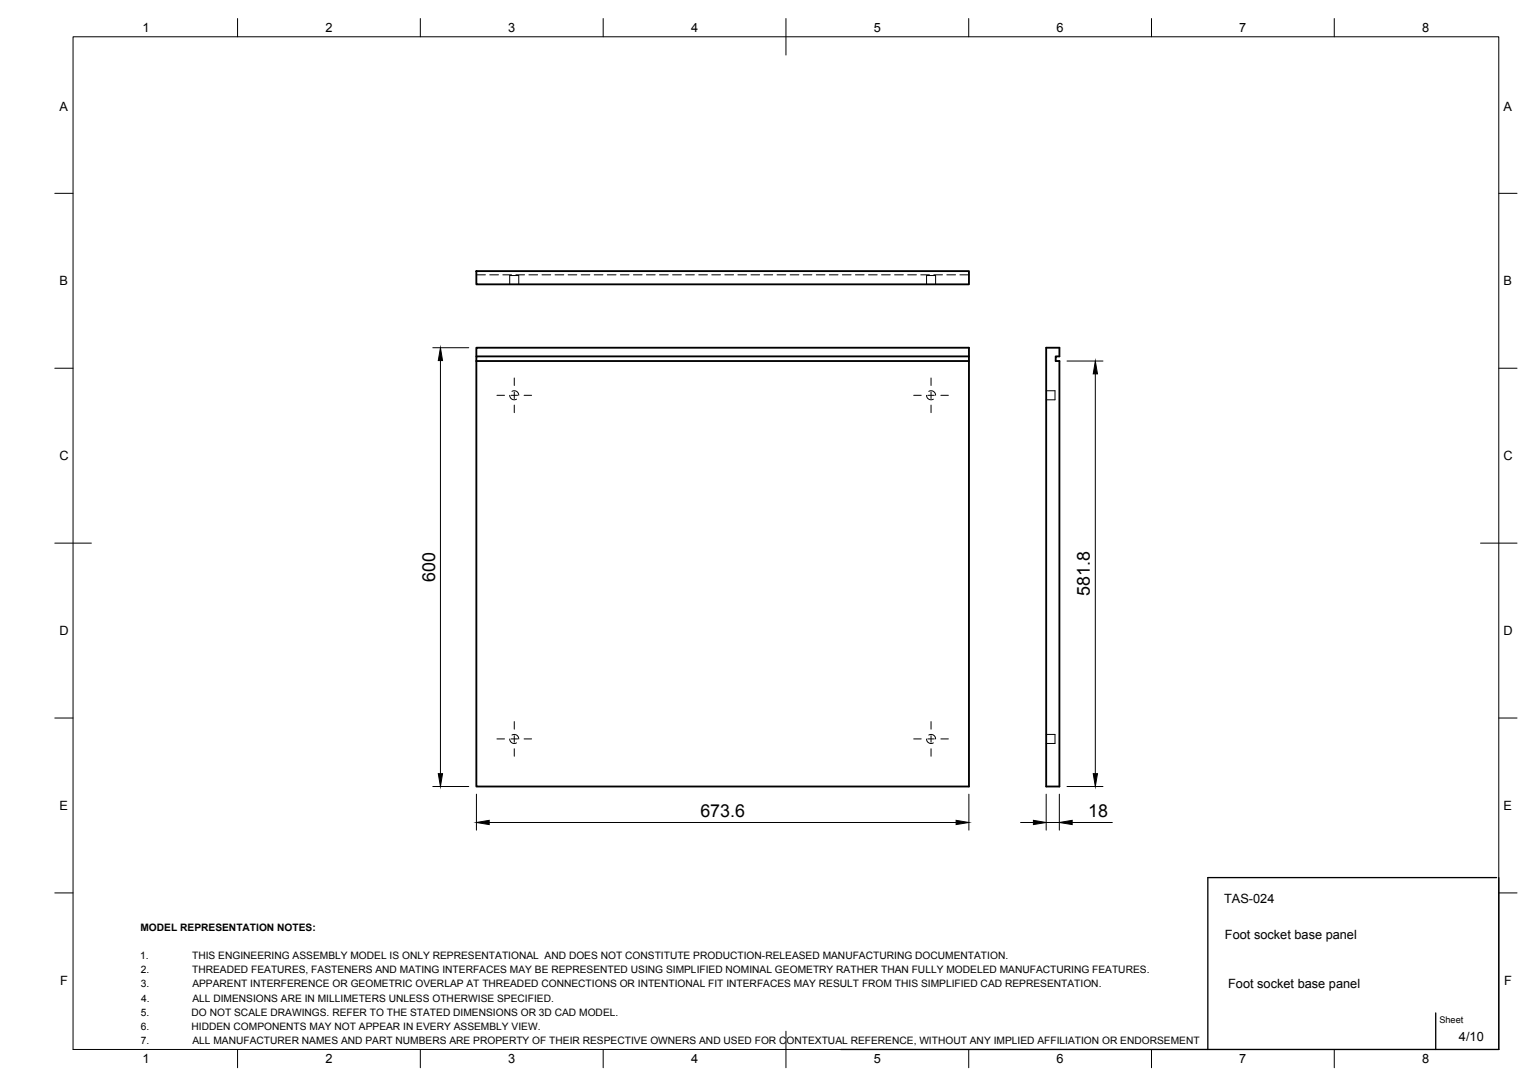
ISO-10303-21;
HEADER;
/* Generated by software containing ST-Developer
 * from STEP Tools, Inc. (www.steptools.com) 
 */

FILE_DESCRIPTION(
/* description */ (''),
/* implementation_level */ '2;1');

FILE_NAME(
/* name */ 'Foot socket base panel.step',
/* time_stamp */ '2026-11-15T17:53:25-08:00',
/* author */ (''),
/* organization */ (''),
/* preprocessor_version */ 'ST-DEVELOPER v20.2',
/* originating_system */ 'Autodesk Translation Framework v15.17.0.0',
/* authorisation */ '');

FILE_SCHEMA (('AUTOMOTIVE_DESIGN { 1 0 10303 214 3 1 1 }'));
ENDSEC;

DATA;
#10=MECHANICAL_DESIGN_GEOMETRIC_PRESENTATION_REPRESENTATION('',(#132),#2673);
#116=SHAPE_REPRESENTATION_RELATIONSHIP('SRR','None',#2724,#124);
#124=ADVANCED_BREP_SHAPE_REPRESENTATION('',(#140),#2666);
#132=STYLED_ITEM('',(#2773),#140);
#140=MANIFOLD_SOLID_BREP('Body1',#1518);
#153=FACE_BOUND('',#380,.T.);
#154=FACE_BOUND('',#381,.T.);
#155=FACE_BOUND('',#382,.T.);
#156=FACE_BOUND('',#383,.T.);
#188=PLANE('',#1666);
#189=PLANE('',#1670);
#190=PLANE('',#1674);
#191=PLANE('',#1678);
#192=PLANE('',#1679);
#193=PLANE('',#1680);
#194=PLANE('',#1681);
#195=PLANE('',#1682);
#196=PLANE('',#1683);
#197=PLANE('',#1684);
#198=PLANE('',#1685);
#199=PLANE('',#1686);
#200=PLANE('',#1687);
#201=PLANE('',#1688);
#267=FACE_OUTER_BOUND('',#362,.T.);
#268=FACE_OUTER_BOUND('',#363,.T.);
#269=FACE_OUTER_BOUND('',#364,.T.);
#270=FACE_OUTER_BOUND('',#365,.T.);
#271=FACE_OUTER_BOUND('',#366,.T.);
#272=FACE_OUTER_BOUND('',#367,.T.);
#273=FACE_OUTER_BOUND('',#368,.T.);
#274=FACE_OUTER_BOUND('',#369,.T.);
#275=FACE_OUTER_BOUND('',#370,.T.);
#276=FACE_OUTER_BOUND('',#371,.T.);
#277=FACE_OUTER_BOUND('',#372,.T.);
#278=FACE_OUTER_BOUND('',#373,.T.);
#279=FACE_OUTER_BOUND('',#374,.T.);
#280=FACE_OUTER_BOUND('',#375,.T.);
#281=FACE_OUTER_BOUND('',#376,.T.);
#282=FACE_OUTER_BOUND('',#377,.T.);
#283=FACE_OUTER_BOUND('',#378,.T.);
#284=FACE_OUTER_BOUND('',#379,.T.);
#362=EDGE_LOOP('',(#1208,#1209,#1210,#1211));
#363=EDGE_LOOP('',(#1212));
#364=EDGE_LOOP('',(#1213,#1214,#1215,#1216));
#365=EDGE_LOOP('',(#1217));
#366=EDGE_LOOP('',(#1218,#1219,#1220,#1221));
#367=EDGE_LOOP('',(#1222));
#368=EDGE_LOOP('',(#1223,#1224,#1225,#1226));
#369=EDGE_LOOP('',(#1227));
#370=EDGE_LOOP('',(#1228,#1229,#1230,#1231));
#371=EDGE_LOOP('',(#1232,#1233,#1234,#1235));
#372=EDGE_LOOP('',(#1236,#1237,#1238,#1239));
#373=EDGE_LOOP('',(#1240,#1241,#1242,#1243,#1244,#1245,#1246,#1247));
#374=EDGE_LOOP('',(#1248,#1249,#1250,#1251));
#375=EDGE_LOOP('',(#1252,#1253,#1254,#1255));
#376=EDGE_LOOP('',(#1256,#1257,#1258,#1259));
#377=EDGE_LOOP('',(#1260,#1261,#1262,#1263,#1264,#1265,#1266,#1267));
#378=EDGE_LOOP('',(#1268,#1269,#1270,#1271));
#379=EDGE_LOOP('',(#1272,#1273,#1274,#1275));
#380=EDGE_LOOP('',(#1276));
#381=EDGE_LOOP('',(#1277));
#382=EDGE_LOOP('',(#1278));
#383=EDGE_LOOP('',(#1279));
#490=LINE('',#2401,#638);
#491=LINE('',#2408,#639);
#492=LINE('',#2415,#640);
#493=LINE('',#2422,#641);
#494=LINE('',#2428,#642);
#495=LINE('',#2430,#643);
#496=LINE('',#2432,#644);
#497=LINE('',#2433,#645);
#498=LINE('',#2437,#646);
#499=LINE('',#2439,#647);
#500=LINE('',#2441,#648);
#501=LINE('',#2442,#649);
#502=LINE('',#2444,#650);
#503=LINE('',#2445,#651);
#504=LINE('',#2448,#652);
#505=LINE('',#2450,#653);
#506=LINE('',#2452,#654);
#507=LINE('',#2454,#655);
#508=LINE('',#2455,#656);
#509=LINE('',#2458,#657);
#510=LINE('',#2459,#658);
#511=LINE('',#2462,#659);
#512=LINE('',#2464,#660);
#513=LINE('',#2465,#661);
#514=LINE('',#2468,#662);
#515=LINE('',#2469,#663);
#516=LINE('',#2471,#664);
#517=LINE('',#2472,#665);
#638=VECTOR('',#1938,0.619999999999997);
#639=VECTOR('',#1947,0.62);
#640=VECTOR('',#1956,0.62);
#641=VECTOR('',#1965,0.619999999999997);
#642=VECTOR('',#1972,1.);
#643=VECTOR('',#1973,1.);
#644=VECTOR('',#1974,1.);
#645=VECTOR('',#1975,1.);
#646=VECTOR('',#1978,1.);
#647=VECTOR('',#1979,1.);
#648=VECTOR('',#1980,1.);
#649=VECTOR('',#1981,1.);
#650=VECTOR('',#1984,1.);
#651=VECTOR('',#1985,1.);
#652=VECTOR('',#1988,1.);
#653=VECTOR('',#1989,1.);
#654=VECTOR('',#1990,1.);
#655=VECTOR('',#1991,1.);
#656=VECTOR('',#1992,1.);
#657=VECTOR('',#1995,1.);
#658=VECTOR('',#1996,1.);
#659=VECTOR('',#1999,1.);
#660=VECTOR('',#2000,1.);
#661=VECTOR('',#2001,1.);
#662=VECTOR('',#2004,1.);
#663=VECTOR('',#2005,1.);
#664=VECTOR('',#2008,1.);
#665=VECTOR('',#2009,1.);
#732=CIRCLE('',#1664,0.619999999999997);
#733=CIRCLE('',#1665,0.619999999999997);
#734=CIRCLE('',#1668,0.62);
#735=CIRCLE('',#1669,0.62);
#736=CIRCLE('',#1672,0.62);
#737=CIRCLE('',#1673,0.62);
#738=CIRCLE('',#1676,0.619999999999997);
#739=CIRCLE('',#1677,0.619999999999997);
#804=VERTEX_POINT('',#2398);
#805=VERTEX_POINT('',#2400);
#806=VERTEX_POINT('',#2405);
#807=VERTEX_POINT('',#2407);
#808=VERTEX_POINT('',#2412);
#809=VERTEX_POINT('',#2414);
#810=VERTEX_POINT('',#2419);
#811=VERTEX_POINT('',#2421);
#812=VERTEX_POINT('',#2426);
#813=VERTEX_POINT('',#2427);
#814=VERTEX_POINT('',#2429);
#815=VERTEX_POINT('',#2431);
#816=VERTEX_POINT('',#2435);
#817=VERTEX_POINT('',#2436);
#818=VERTEX_POINT('',#2438);
#819=VERTEX_POINT('',#2440);
#820=VERTEX_POINT('',#2447);
#821=VERTEX_POINT('',#2449);
#822=VERTEX_POINT('',#2451);
#823=VERTEX_POINT('',#2453);
#824=VERTEX_POINT('',#2457);
#825=VERTEX_POINT('',#2461);
#826=VERTEX_POINT('',#2463);
#827=VERTEX_POINT('',#2467);
#950=EDGE_CURVE('',#804,#804,#732,.T.);
#951=EDGE_CURVE('',#804,#805,#490,.T.);
#952=EDGE_CURVE('',#805,#805,#733,.T.);
#953=EDGE_CURVE('',#806,#806,#734,.T.);
#954=EDGE_CURVE('',#806,#807,#491,.T.);
#955=EDGE_CURVE('',#807,#807,#735,.T.);
#956=EDGE_CURVE('',#808,#808,#736,.T.);
#957=EDGE_CURVE('',#808,#809,#492,.T.);
#958=EDGE_CURVE('',#809,#809,#737,.T.);
#959=EDGE_CURVE('',#810,#810,#738,.T.);
#960=EDGE_CURVE('',#810,#811,#493,.T.);
#961=EDGE_CURVE('',#811,#811,#739,.T.);
#962=EDGE_CURVE('',#812,#813,#494,.T.);
#963=EDGE_CURVE('',#814,#812,#495,.T.);
#964=EDGE_CURVE('',#815,#814,#496,.T.);
#965=EDGE_CURVE('',#813,#815,#497,.T.);
#966=EDGE_CURVE('',#816,#817,#498,.T.);
#967=EDGE_CURVE('',#818,#816,#499,.T.);
#968=EDGE_CURVE('',#819,#818,#500,.T.);
#969=EDGE_CURVE('',#817,#819,#501,.T.);
#970=EDGE_CURVE('',#815,#818,#502,.T.);
#971=EDGE_CURVE('',#819,#814,#503,.T.);
#972=EDGE_CURVE('',#820,#812,#504,.T.);
#973=EDGE_CURVE('',#821,#820,#505,.T.);
#974=EDGE_CURVE('',#821,#822,#506,.T.);
#975=EDGE_CURVE('',#822,#823,#507,.T.);
#976=EDGE_CURVE('',#817,#823,#508,.T.);
#977=EDGE_CURVE('',#813,#824,#509,.T.);
#978=EDGE_CURVE('',#824,#820,#510,.T.);
#979=EDGE_CURVE('',#822,#825,#511,.T.);
#980=EDGE_CURVE('',#825,#826,#512,.T.);
#981=EDGE_CURVE('',#823,#826,#513,.T.);
#982=EDGE_CURVE('',#827,#821,#514,.T.);
#983=EDGE_CURVE('',#827,#824,#515,.T.);
#984=EDGE_CURVE('',#826,#816,#516,.T.);
#985=EDGE_CURVE('',#825,#827,#517,.T.);
#1208=ORIENTED_EDGE('',*,*,#950,.F.);
#1209=ORIENTED_EDGE('',*,*,#951,.T.);
#1210=ORIENTED_EDGE('',*,*,#952,.T.);
#1211=ORIENTED_EDGE('',*,*,#951,.F.);
#1212=ORIENTED_EDGE('',*,*,#952,.F.);
#1213=ORIENTED_EDGE('',*,*,#953,.F.);
#1214=ORIENTED_EDGE('',*,*,#954,.T.);
#1215=ORIENTED_EDGE('',*,*,#955,.T.);
#1216=ORIENTED_EDGE('',*,*,#954,.F.);
#1217=ORIENTED_EDGE('',*,*,#955,.F.);
#1218=ORIENTED_EDGE('',*,*,#956,.F.);
#1219=ORIENTED_EDGE('',*,*,#957,.T.);
#1220=ORIENTED_EDGE('',*,*,#958,.T.);
#1221=ORIENTED_EDGE('',*,*,#957,.F.);
#1222=ORIENTED_EDGE('',*,*,#958,.F.);
#1223=ORIENTED_EDGE('',*,*,#959,.F.);
#1224=ORIENTED_EDGE('',*,*,#960,.T.);
#1225=ORIENTED_EDGE('',*,*,#961,.T.);
#1226=ORIENTED_EDGE('',*,*,#960,.F.);
#1227=ORIENTED_EDGE('',*,*,#961,.F.);
#1228=ORIENTED_EDGE('',*,*,#962,.F.);
#1229=ORIENTED_EDGE('',*,*,#963,.F.);
#1230=ORIENTED_EDGE('',*,*,#964,.F.);
#1231=ORIENTED_EDGE('',*,*,#965,.F.);
#1232=ORIENTED_EDGE('',*,*,#966,.F.);
#1233=ORIENTED_EDGE('',*,*,#967,.F.);
#1234=ORIENTED_EDGE('',*,*,#968,.F.);
#1235=ORIENTED_EDGE('',*,*,#969,.F.);
#1236=ORIENTED_EDGE('',*,*,#970,.F.);
#1237=ORIENTED_EDGE('',*,*,#964,.T.);
#1238=ORIENTED_EDGE('',*,*,#971,.F.);
#1239=ORIENTED_EDGE('',*,*,#968,.T.);
#1240=ORIENTED_EDGE('',*,*,#969,.T.);
#1241=ORIENTED_EDGE('',*,*,#971,.T.);
#1242=ORIENTED_EDGE('',*,*,#963,.T.);
#1243=ORIENTED_EDGE('',*,*,#972,.F.);
#1244=ORIENTED_EDGE('',*,*,#973,.F.);
#1245=ORIENTED_EDGE('',*,*,#974,.T.);
#1246=ORIENTED_EDGE('',*,*,#975,.T.);
#1247=ORIENTED_EDGE('',*,*,#976,.F.);
#1248=ORIENTED_EDGE('',*,*,#962,.T.);
#1249=ORIENTED_EDGE('',*,*,#977,.T.);
#1250=ORIENTED_EDGE('',*,*,#978,.T.);
#1251=ORIENTED_EDGE('',*,*,#972,.T.);
#1252=ORIENTED_EDGE('',*,*,#979,.T.);
#1253=ORIENTED_EDGE('',*,*,#980,.T.);
#1254=ORIENTED_EDGE('',*,*,#981,.F.);
#1255=ORIENTED_EDGE('',*,*,#975,.F.);
#1256=ORIENTED_EDGE('',*,*,#982,.T.);
#1257=ORIENTED_EDGE('',*,*,#973,.T.);
#1258=ORIENTED_EDGE('',*,*,#978,.F.);
#1259=ORIENTED_EDGE('',*,*,#983,.F.);
#1260=ORIENTED_EDGE('',*,*,#967,.T.);
#1261=ORIENTED_EDGE('',*,*,#984,.F.);
#1262=ORIENTED_EDGE('',*,*,#980,.F.);
#1263=ORIENTED_EDGE('',*,*,#985,.T.);
#1264=ORIENTED_EDGE('',*,*,#983,.T.);
#1265=ORIENTED_EDGE('',*,*,#977,.F.);
#1266=ORIENTED_EDGE('',*,*,#965,.T.);
#1267=ORIENTED_EDGE('',*,*,#970,.T.);
#1268=ORIENTED_EDGE('',*,*,#966,.T.);
#1269=ORIENTED_EDGE('',*,*,#976,.T.);
#1270=ORIENTED_EDGE('',*,*,#981,.T.);
#1271=ORIENTED_EDGE('',*,*,#984,.T.);
#1272=ORIENTED_EDGE('',*,*,#985,.F.);
#1273=ORIENTED_EDGE('',*,*,#979,.F.);
#1274=ORIENTED_EDGE('',*,*,#974,.F.);
#1275=ORIENTED_EDGE('',*,*,#982,.F.);
#1276=ORIENTED_EDGE('',*,*,#950,.T.);
#1277=ORIENTED_EDGE('',*,*,#953,.T.);
#1278=ORIENTED_EDGE('',*,*,#956,.T.);
#1279=ORIENTED_EDGE('',*,*,#959,.T.);
#1418=CYLINDRICAL_SURFACE('',#1663,0.619999999999997);
#1419=CYLINDRICAL_SURFACE('',#1667,0.62);
#1420=CYLINDRICAL_SURFACE('',#1671,0.62);
#1421=CYLINDRICAL_SURFACE('',#1675,0.619999999999997);
#1462=ADVANCED_FACE('',(#267),#1418,.F.);
#1463=ADVANCED_FACE('',(#268),#188,.F.);
#1464=ADVANCED_FACE('',(#269),#1419,.F.);
#1465=ADVANCED_FACE('',(#270),#189,.F.);
#1466=ADVANCED_FACE('',(#271),#1420,.F.);
#1467=ADVANCED_FACE('',(#272),#190,.F.);
#1468=ADVANCED_FACE('',(#273),#1421,.F.);
#1469=ADVANCED_FACE('',(#274),#191,.F.);
#1470=ADVANCED_FACE('',(#275),#192,.F.);
#1471=ADVANCED_FACE('',(#276),#193,.F.);
#1472=ADVANCED_FACE('',(#277),#194,.T.);
#1473=ADVANCED_FACE('',(#278),#195,.T.);
#1474=ADVANCED_FACE('',(#279),#196,.T.);
#1475=ADVANCED_FACE('',(#280),#197,.T.);
#1476=ADVANCED_FACE('',(#281),#198,.T.);
#1477=ADVANCED_FACE('',(#282),#199,.T.);
#1478=ADVANCED_FACE('',(#283),#200,.T.);
#1479=ADVANCED_FACE('',(#284,#153,#154,#155,#156),#201,.F.);
#1518=CLOSED_SHELL('',(#1462,#1463,#1464,#1465,#1466,#1467,#1468,#1469,
#1470,#1471,#1472,#1473,#1474,#1475,#1476,#1477,#1478,#1479));
#1662=AXIS2_PLACEMENT_3D('',#2396,#1932,#1933);
#1663=AXIS2_PLACEMENT_3D('',#2397,#1934,#1935);
#1664=AXIS2_PLACEMENT_3D('',#2399,#1936,#1937);
#1665=AXIS2_PLACEMENT_3D('',#2402,#1939,#1940);
#1666=AXIS2_PLACEMENT_3D('',#2403,#1941,#1942);
#1667=AXIS2_PLACEMENT_3D('',#2404,#1943,#1944);
#1668=AXIS2_PLACEMENT_3D('',#2406,#1945,#1946);
#1669=AXIS2_PLACEMENT_3D('',#2409,#1948,#1949);
#1670=AXIS2_PLACEMENT_3D('',#2410,#1950,#1951);
#1671=AXIS2_PLACEMENT_3D('',#2411,#1952,#1953);
#1672=AXIS2_PLACEMENT_3D('',#2413,#1954,#1955);
#1673=AXIS2_PLACEMENT_3D('',#2416,#1957,#1958);
#1674=AXIS2_PLACEMENT_3D('',#2417,#1959,#1960);
#1675=AXIS2_PLACEMENT_3D('',#2418,#1961,#1962);
#1676=AXIS2_PLACEMENT_3D('',#2420,#1963,#1964);
#1677=AXIS2_PLACEMENT_3D('',#2423,#1966,#1967);
#1678=AXIS2_PLACEMENT_3D('',#2424,#1968,#1969);
#1679=AXIS2_PLACEMENT_3D('',#2425,#1970,#1971);
#1680=AXIS2_PLACEMENT_3D('',#2434,#1976,#1977);
#1681=AXIS2_PLACEMENT_3D('',#2443,#1982,#1983);
#1682=AXIS2_PLACEMENT_3D('',#2446,#1986,#1987);
#1683=AXIS2_PLACEMENT_3D('',#2456,#1993,#1994);
#1684=AXIS2_PLACEMENT_3D('',#2460,#1997,#1998);
#1685=AXIS2_PLACEMENT_3D('',#2466,#2002,#2003);
#1686=AXIS2_PLACEMENT_3D('',#2470,#2006,#2007);
#1687=AXIS2_PLACEMENT_3D('',#2473,#2010,#2011);
#1688=AXIS2_PLACEMENT_3D('',#2474,#2012,#2013);
#1932=DIRECTION('axis',(0.,0.,1.));
#1933=DIRECTION('refdir',(1.,0.,0.));
#1934=DIRECTION('center_axis',(0.,0.,1.));
#1935=DIRECTION('ref_axis',(1.,0.,0.));
#1936=DIRECTION('center_axis',(0.,0.,1.));
#1937=DIRECTION('ref_axis',(1.,0.,0.));
#1938=DIRECTION('',(0.,0.,1.));
#1939=DIRECTION('center_axis',(0.,0.,1.));
#1940=DIRECTION('ref_axis',(1.,0.,0.));
#1941=DIRECTION('center_axis',(0.,0.,1.));
#1942=DIRECTION('ref_axis',(1.,0.,0.));
#1943=DIRECTION('center_axis',(0.,0.,1.));
#1944=DIRECTION('ref_axis',(1.,0.,0.));
#1945=DIRECTION('center_axis',(0.,0.,1.));
#1946=DIRECTION('ref_axis',(1.,0.,0.));
#1947=DIRECTION('',(0.,0.,1.));
#1948=DIRECTION('center_axis',(0.,0.,1.));
#1949=DIRECTION('ref_axis',(1.,0.,0.));
#1950=DIRECTION('center_axis',(0.,0.,1.));
#1951=DIRECTION('ref_axis',(1.,0.,0.));
#1952=DIRECTION('center_axis',(0.,0.,1.));
#1953=DIRECTION('ref_axis',(1.,0.,0.));
#1954=DIRECTION('center_axis',(0.,0.,1.));
#1955=DIRECTION('ref_axis',(1.,0.,0.));
#1956=DIRECTION('',(0.,0.,1.));
#1957=DIRECTION('center_axis',(0.,0.,1.));
#1958=DIRECTION('ref_axis',(1.,0.,0.));
#1959=DIRECTION('center_axis',(0.,0.,1.));
#1960=DIRECTION('ref_axis',(1.,0.,0.));
#1961=DIRECTION('center_axis',(0.,0.,1.));
#1962=DIRECTION('ref_axis',(1.,0.,0.));
#1963=DIRECTION('center_axis',(0.,0.,1.));
#1964=DIRECTION('ref_axis',(1.,0.,0.));
#1965=DIRECTION('',(0.,0.,1.));
#1966=DIRECTION('center_axis',(0.,0.,1.));
#1967=DIRECTION('ref_axis',(1.,0.,0.));
#1968=DIRECTION('center_axis',(0.,0.,1.));
#1969=DIRECTION('ref_axis',(1.,0.,0.));
#1970=DIRECTION('center_axis',(0.,-1.,0.));
#1971=DIRECTION('ref_axis',(1.,0.,0.));
#1972=DIRECTION('',(-1.,0.,0.));
#1973=DIRECTION('',(0.,0.,1.));
#1974=DIRECTION('',(1.,0.,0.));
#1975=DIRECTION('',(0.,0.,-1.));
#1976=DIRECTION('center_axis',(0.,1.,0.));
#1977=DIRECTION('ref_axis',(-1.,0.,0.));
#1978=DIRECTION('',(1.,0.,0.));
#1979=DIRECTION('',(0.,0.,1.));
#1980=DIRECTION('',(-1.,0.,0.));
#1981=DIRECTION('',(0.,0.,-1.));
#1982=DIRECTION('center_axis',(0.,0.,1.));
#1983=DIRECTION('ref_axis',(1.,0.,0.));
#1984=DIRECTION('',(0.,1.,0.));
#1985=DIRECTION('',(0.,-1.,0.));
#1986=DIRECTION('center_axis',(1.,0.,0.));
#1987=DIRECTION('ref_axis',(0.,1.,0.));
#1988=DIRECTION('',(0.,1.,0.));
#1989=DIRECTION('',(0.,0.,1.));
#1990=DIRECTION('',(0.,1.,0.));
#1991=DIRECTION('',(0.,0.,1.));
#1992=DIRECTION('',(0.,1.,0.));
#1993=DIRECTION('center_axis',(0.,0.,1.));
#1994=DIRECTION('ref_axis',(1.,0.,0.));
#1995=DIRECTION('',(0.,-1.,0.));
#1996=DIRECTION('',(1.,0.,0.));
#1997=DIRECTION('center_axis',(0.,1.,0.));
#1998=DIRECTION('ref_axis',(-1.,0.,0.));
#1999=DIRECTION('',(-1.,0.,0.));
#2000=DIRECTION('',(0.,0.,1.));
#2001=DIRECTION('',(-1.,0.,0.));
#2002=DIRECTION('center_axis',(0.,-1.,0.));
#2003=DIRECTION('ref_axis',(1.,0.,0.));
#2004=DIRECTION('',(1.,0.,0.));
#2005=DIRECTION('',(0.,0.,1.));
#2006=DIRECTION('center_axis',(-1.,0.,0.));
#2007=DIRECTION('ref_axis',(0.,-1.,0.));
#2008=DIRECTION('',(0.,-1.,0.));
#2009=DIRECTION('',(0.,-1.,0.));
#2010=DIRECTION('center_axis',(0.,0.,1.));
#2011=DIRECTION('ref_axis',(1.,0.,0.));
#2012=DIRECTION('center_axis',(0.,0.,1.));
#2013=DIRECTION('ref_axis',(1.,0.,0.));
#2396=CARTESIAN_POINT('',(0.,0.,0.));
#2397=CARTESIAN_POINT('Origin',(62.18,6.5,0.));
#2398=CARTESIAN_POINT('',(61.56,6.5,0.));
#2399=CARTESIAN_POINT('Origin',(62.18,6.5,0.));
#2400=CARTESIAN_POINT('',(61.56,6.5,1.2));
#2401=CARTESIAN_POINT('',(61.56,6.5,0.));
#2402=CARTESIAN_POINT('Origin',(62.18,6.5,1.2));
#2403=CARTESIAN_POINT('Origin',(62.18,6.5,1.2));
#2404=CARTESIAN_POINT('Origin',(5.18,53.5,0.));
#2405=CARTESIAN_POINT('',(4.56,53.5,0.));
#2406=CARTESIAN_POINT('Origin',(5.18,53.5,0.));
#2407=CARTESIAN_POINT('',(4.56,53.5,1.2));
#2408=CARTESIAN_POINT('',(4.56,53.5,0.));
#2409=CARTESIAN_POINT('Origin',(5.18,53.5,1.2));
#2410=CARTESIAN_POINT('Origin',(5.18,53.5,1.2));
#2411=CARTESIAN_POINT('Origin',(5.18,6.5,0.));
#2412=CARTESIAN_POINT('',(4.56,6.5,0.));
#2413=CARTESIAN_POINT('Origin',(5.18,6.5,0.));
#2414=CARTESIAN_POINT('',(4.56,6.5,1.2));
#2415=CARTESIAN_POINT('',(4.56,6.5,0.));
#2416=CARTESIAN_POINT('Origin',(5.18,6.5,1.2));
#2417=CARTESIAN_POINT('Origin',(5.18,6.5,1.2));
#2418=CARTESIAN_POINT('Origin',(62.18,53.5,0.));
#2419=CARTESIAN_POINT('',(61.56,53.5,0.));
#2420=CARTESIAN_POINT('Origin',(62.18,53.5,0.));
#2421=CARTESIAN_POINT('',(61.56,53.5,1.2));
#2422=CARTESIAN_POINT('',(61.56,53.5,0.));
#2423=CARTESIAN_POINT('Origin',(62.18,53.5,1.2));
#2424=CARTESIAN_POINT('Origin',(62.18,53.5,1.2));
#2425=CARTESIAN_POINT('Origin',(0.,58.18,1.3));
#2426=CARTESIAN_POINT('',(67.36,58.18,1.8));
#2427=CARTESIAN_POINT('',(0.,58.18,1.8));
#2428=CARTESIAN_POINT('',(16.84,58.18,1.8));
#2429=CARTESIAN_POINT('',(67.36,58.18,1.3));
#2430=CARTESIAN_POINT('',(67.36,58.18,0.65));
#2431=CARTESIAN_POINT('',(0.,58.18,1.3));
#2432=CARTESIAN_POINT('',(0.,58.18,1.3));
#2433=CARTESIAN_POINT('',(0.,58.18,0.65));
#2434=CARTESIAN_POINT('Origin',(67.36,58.82,1.3));
#2435=CARTESIAN_POINT('',(0.,58.82,1.8));
#2436=CARTESIAN_POINT('',(67.36,58.82,1.8));
#2437=CARTESIAN_POINT('',(50.52,58.82,1.8));
#2438=CARTESIAN_POINT('',(0.,58.82,1.3));
#2439=CARTESIAN_POINT('',(0.,58.82,0.65));
#2440=CARTESIAN_POINT('',(67.36,58.82,1.3));
#2441=CARTESIAN_POINT('',(67.36,58.82,1.3));
#2442=CARTESIAN_POINT('',(67.36,58.82,0.65));
#2443=CARTESIAN_POINT('Origin',(33.68,58.5,1.3));
#2444=CARTESIAN_POINT('',(0.,59.25,1.3));
#2445=CARTESIAN_POINT('',(67.36,29.25,1.3));
#2446=CARTESIAN_POINT('Origin',(67.36,0.,0.));
#2447=CARTESIAN_POINT('',(67.36,0.,1.8));
#2448=CARTESIAN_POINT('',(67.36,0.,1.8));
#2449=CARTESIAN_POINT('',(67.36,0.,0.));
#2450=CARTESIAN_POINT('',(67.36,0.,0.));
#2451=CARTESIAN_POINT('',(67.36,60.,0.));
#2452=CARTESIAN_POINT('',(67.36,0.,0.));
#2453=CARTESIAN_POINT('',(67.36,60.,1.8));
#2454=CARTESIAN_POINT('',(67.36,60.,0.));
#2455=CARTESIAN_POINT('',(67.36,0.,1.8));
#2456=CARTESIAN_POINT('Origin',(33.68,30.,1.8));
#2457=CARTESIAN_POINT('',(0.,0.,1.8));
#2458=CARTESIAN_POINT('',(0.,60.,1.8));
#2459=CARTESIAN_POINT('',(0.,0.,1.8));
#2460=CARTESIAN_POINT('Origin',(67.36,60.,0.));
#2461=CARTESIAN_POINT('',(0.,60.,0.));
#2462=CARTESIAN_POINT('',(67.36,60.,0.));
#2463=CARTESIAN_POINT('',(0.,60.,1.8));
#2464=CARTESIAN_POINT('',(0.,60.,0.));
#2465=CARTESIAN_POINT('',(67.36,60.,1.8));
#2466=CARTESIAN_POINT('Origin',(0.,0.,0.));
#2467=CARTESIAN_POINT('',(0.,0.,0.));
#2468=CARTESIAN_POINT('',(0.,0.,0.));
#2469=CARTESIAN_POINT('',(0.,0.,0.));
#2470=CARTESIAN_POINT('Origin',(0.,60.,0.));
#2471=CARTESIAN_POINT('',(0.,60.,1.8));
#2472=CARTESIAN_POINT('',(0.,60.,0.));
#2473=CARTESIAN_POINT('Origin',(33.68,30.,1.8));
#2474=CARTESIAN_POINT('Origin',(33.68,30.,0.));
#2656=UNCERTAINTY_MEASURE_WITH_UNIT(LENGTH_MEASURE(0.001),#2674,
'DISTANCE_ACCURACY_VALUE',
'Maximum model space distance between geometric entities at asserted c
onnectivities');
#2663=UNCERTAINTY_MEASURE_WITH_UNIT(LENGTH_MEASURE(0.001),#2674,
'DISTANCE_ACCURACY_VALUE',
'Maximum model space distance between geometric entities at asserted c
onnectivities');
#2666=(
GEOMETRIC_REPRESENTATION_CONTEXT(3)
GLOBAL_UNCERTAINTY_ASSIGNED_CONTEXT((#2656))
GLOBAL_UNIT_ASSIGNED_CONTEXT((#2674,#2676,#2677))
REPRESENTATION_CONTEXT('','3D')
);
#2673=(
GEOMETRIC_REPRESENTATION_CONTEXT(3)
GLOBAL_UNCERTAINTY_ASSIGNED_CONTEXT((#2663))
GLOBAL_UNIT_ASSIGNED_CONTEXT((#2674,#2676,#2677))
REPRESENTATION_CONTEXT('','3D')
);
#2674=(
LENGTH_UNIT()
NAMED_UNIT(*)
SI_UNIT(.CENTI.,.METRE.)
);
#2676=(
NAMED_UNIT(*)
PLANE_ANGLE_UNIT()
SI_UNIT($,.RADIAN.)
);
#2677=(
NAMED_UNIT(*)
SI_UNIT($,.STERADIAN.)
SOLID_ANGLE_UNIT()
);
#2680=SHAPE_DEFINITION_REPRESENTATION(#2689,#2724);
#2689=PRODUCT_DEFINITION_SHAPE('',$,#2734);
#2724=SHAPE_REPRESENTATION('',(#1662),#2666);
#2731=PRODUCT_DEFINITION_CONTEXT('part definition',#2760,'design');
#2734=PRODUCT_DEFINITION('Foot socket base panel',
'Foot socket base panel',#2743,#2731);
#2743=PRODUCT_DEFINITION_FORMATION('',$,#2764);
#2760=APPLICATION_CONTEXT(
'Core Data for Automotive Mechanical Design Process');
#2761=PRODUCT_CONTEXT('part definition',#2760,'mechanical');
#2764=PRODUCT('Foot socket base panel','Foot socket base panel',$,(#2761));
#2773=PRESENTATION_STYLE_ASSIGNMENT((#2782));
#2782=SURFACE_STYLE_USAGE(.BOTH.,#2791);
#2791=SURFACE_SIDE_STYLE('',(#2800));
#2800=SURFACE_STYLE_FILL_AREA(#2809);
#2809=FILL_AREA_STYLE('Foot socket base panel finish',(#2818));
#2818=FILL_AREA_STYLE_COLOUR('Foot socket base panel finish',#2827);
#2827=COLOUR_RGB('Foot socket base panel finish',0.662745098039216,0.823529411764706,
0.917647058823529);
ENDSEC;
END-ISO-10303-21;
